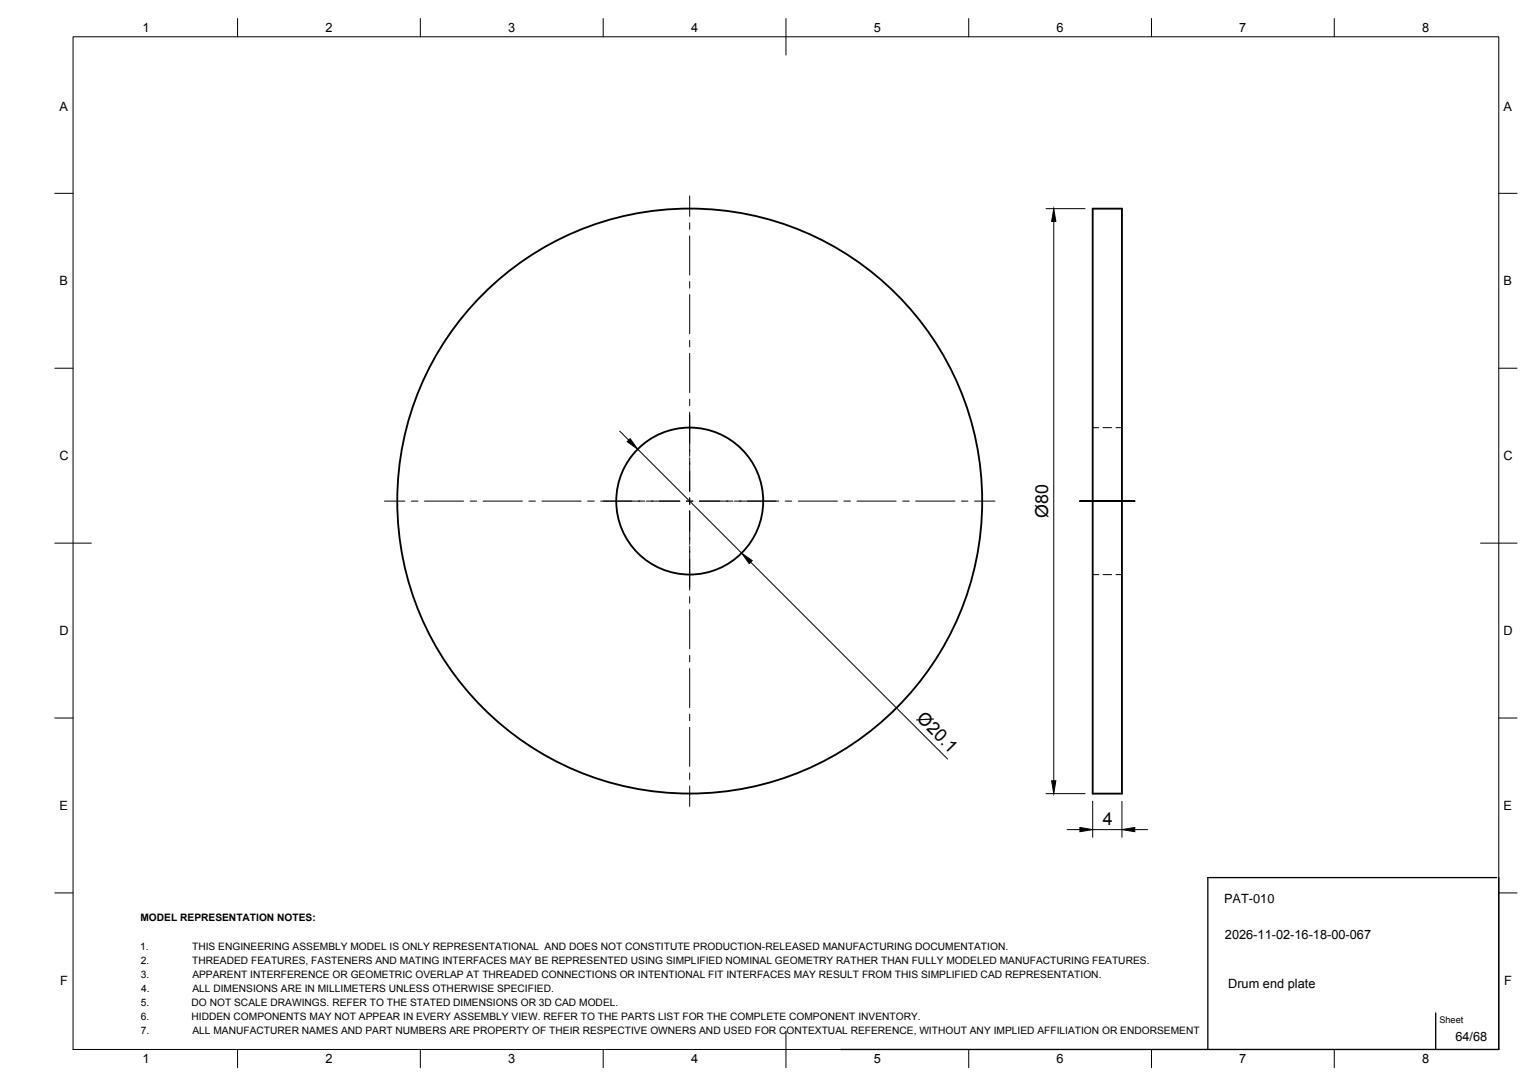
ISO-10303-21;
HEADER;
/* Generated by software containing ST-Developer
 * from STEP Tools, Inc. (www.steptools.com) 
 */

FILE_DESCRIPTION(
/* description */ ('Belt conveyor head drive unit'),
/* implementation_level */ '2;1');

FILE_NAME(
/* name */ 'Drum end plate.step',
/* time_stamp */ '2026-10-28T03:26:19-07:00',
/* author */ (''),
/* organization */ (''),
/* preprocessor_version */ 'ST-DEVELOPER v20.2',
/* originating_system */ 'Autodesk Translation Framework v15.17.0.0',
/* authorisation */ '');

FILE_SCHEMA (('AUTOMOTIVE_DESIGN { 1 0 10303 214 3 1 1 }'));
ENDSEC;

DATA;
#10=MECHANICAL_DESIGN_GEOMETRIC_PRESENTATION_REPRESENTATION('',(#925),#27069);
#771=SHAPE_REPRESENTATION_RELATIONSHIP('SRR','None',#27420,#840);
#840=ADVANCED_BREP_SHAPE_REPRESENTATION('',(#1006),#27062);
#925=STYLED_ITEM('',(#27790),#1006);
#1006=MANIFOLD_SOLID_BREP('Body1',#13794);
#1252=FACE_BOUND('',#3332,.T.);
#1253=FACE_BOUND('',#3334,.T.);
#1596=PLANE('',#15975);
#1597=PLANE('',#15976);
#2289=FACE_OUTER_BOUND('',#3329,.T.);
#2290=FACE_OUTER_BOUND('',#3330,.T.);
#2291=FACE_OUTER_BOUND('',#3331,.T.);
#2292=FACE_OUTER_BOUND('',#3333,.T.);
#3329=EDGE_LOOP('',(#11770,#11771,#11772,#11773));
#3330=EDGE_LOOP('',(#11774,#11775,#11776,#11777));
#3331=EDGE_LOOP('',(#11778));
#3332=EDGE_LOOP('',(#11779));
#3333=EDGE_LOOP('',(#11780));
#3334=EDGE_LOOP('',(#11781));
#4141=LINE('',#25622,#4933);
#4142=LINE('',#25628,#4934);
#4933=VECTOR('',#19895,1.005);
#4934=VECTOR('',#19902,4.);
#5751=CIRCLE('',#15970,1.005);
#5752=CIRCLE('',#15971,1.005);
#5753=CIRCLE('',#15973,4.);
#5754=CIRCLE('',#15974,4.);
#6915=VERTEX_POINT('',#25619);
#6916=VERTEX_POINT('',#25621);
#6917=VERTEX_POINT('',#25625);
#6918=VERTEX_POINT('',#25627);
#8577=EDGE_CURVE('',#6915,#6915,#5751,.T.);
#8578=EDGE_CURVE('',#6915,#6916,#4141,.T.);
#8579=EDGE_CURVE('',#6916,#6916,#5752,.T.);
#8580=EDGE_CURVE('',#6917,#6917,#5753,.T.);
#8581=EDGE_CURVE('',#6917,#6918,#4142,.T.);
#8582=EDGE_CURVE('',#6918,#6918,#5754,.T.);
#11770=ORIENTED_EDGE('',*,*,#8577,.F.);
#11771=ORIENTED_EDGE('',*,*,#8578,.T.);
#11772=ORIENTED_EDGE('',*,*,#8579,.T.);
#11773=ORIENTED_EDGE('',*,*,#8578,.F.);
#11774=ORIENTED_EDGE('',*,*,#8580,.F.);
#11775=ORIENTED_EDGE('',*,*,#8581,.T.);
#11776=ORIENTED_EDGE('',*,*,#8582,.T.);
#11777=ORIENTED_EDGE('',*,*,#8581,.F.);
#11778=ORIENTED_EDGE('',*,*,#8580,.T.);
#11779=ORIENTED_EDGE('',*,*,#8577,.T.);
#11780=ORIENTED_EDGE('',*,*,#8582,.F.);
#11781=ORIENTED_EDGE('',*,*,#8579,.F.);
#12811=CYLINDRICAL_SURFACE('',#15969,1.005);
#12812=CYLINDRICAL_SURFACE('',#15972,4.);
#13568=ADVANCED_FACE('',(#2289),#12811,.F.);
#13569=ADVANCED_FACE('',(#2290),#12812,.T.);
#13570=ADVANCED_FACE('',(#2291,#1252),#1596,.T.);
#13571=ADVANCED_FACE('',(#2292,#1253),#1597,.F.);
#13794=CLOSED_SHELL('',(#13568,#13569,#13570,#13571));
#15968=AXIS2_PLACEMENT_3D('',#25617,#19889,#19890);
#15969=AXIS2_PLACEMENT_3D('',#25618,#19891,#19892);
#15970=AXIS2_PLACEMENT_3D('',#25620,#19893,#19894);
#15971=AXIS2_PLACEMENT_3D('',#25623,#19896,#19897);
#15972=AXIS2_PLACEMENT_3D('',#25624,#19898,#19899);
#15973=AXIS2_PLACEMENT_3D('',#25626,#19900,#19901);
#15974=AXIS2_PLACEMENT_3D('',#25629,#19903,#19904);
#15975=AXIS2_PLACEMENT_3D('',#25630,#19905,#19906);
#15976=AXIS2_PLACEMENT_3D('',#25631,#19907,#19908);
#19889=DIRECTION('axis',(0.,0.,1.));
#19890=DIRECTION('refdir',(1.,0.,0.));
#19891=DIRECTION('center_axis',(0.,1.,0.));
#19892=DIRECTION('ref_axis',(1.,0.,0.));
#19893=DIRECTION('center_axis',(0.,-1.,0.));
#19894=DIRECTION('ref_axis',(1.,0.,0.));
#19895=DIRECTION('',(0.,-1.,0.));
#19896=DIRECTION('center_axis',(0.,-1.,0.));
#19897=DIRECTION('ref_axis',(1.,0.,0.));
#19898=DIRECTION('center_axis',(0.,1.,0.));
#19899=DIRECTION('ref_axis',(1.,0.,0.));
#19900=DIRECTION('center_axis',(0.,1.,0.));
#19901=DIRECTION('ref_axis',(1.,0.,0.));
#19902=DIRECTION('',(0.,-1.,0.));
#19903=DIRECTION('center_axis',(0.,1.,0.));
#19904=DIRECTION('ref_axis',(1.,0.,0.));
#19905=DIRECTION('center_axis',(0.,1.,0.));
#19906=DIRECTION('ref_axis',(1.,0.,0.));
#19907=DIRECTION('center_axis',(0.,1.,0.));
#19908=DIRECTION('ref_axis',(1.,0.,0.));
#25617=CARTESIAN_POINT('',(0.,0.,0.));
#25618=CARTESIAN_POINT('Origin',(6.97091003018116,6.6,7.));
#25619=CARTESIAN_POINT('',(5.96591003018116,7.,7.));
#25620=CARTESIAN_POINT('Origin',(6.97091003018116,7.,7.));
#25621=CARTESIAN_POINT('',(5.96591003018116,6.6,7.));
#25622=CARTESIAN_POINT('',(5.96591003018116,6.6,7.));
#25623=CARTESIAN_POINT('Origin',(6.97091003018116,6.6,7.));
#25624=CARTESIAN_POINT('Origin',(6.97091003018116,6.6,7.));
#25625=CARTESIAN_POINT('',(2.97091003018116,7.,7.));
#25626=CARTESIAN_POINT('Origin',(6.97091003018116,7.,7.));
#25627=CARTESIAN_POINT('',(2.97091003018116,6.6,7.));
#25628=CARTESIAN_POINT('',(2.97091003018116,6.6,7.));
#25629=CARTESIAN_POINT('Origin',(6.97091003018116,6.6,7.));
#25630=CARTESIAN_POINT('Origin',(6.97091003018116,7.,7.));
#25631=CARTESIAN_POINT('Origin',(6.97091003018116,6.6,7.));
#26985=UNCERTAINTY_MEASURE_WITH_UNIT(LENGTH_MEASURE(0.001),#27070,
'DISTANCE_ACCURACY_VALUE',
'Maximum model space distance between geometric entities at asserted c
onnectivities');
#26992=UNCERTAINTY_MEASURE_WITH_UNIT(LENGTH_MEASURE(0.001),#27070,
'DISTANCE_ACCURACY_VALUE',
'Maximum model space distance between geometric entities at asserted c
onnectivities');
#27062=(
GEOMETRIC_REPRESENTATION_CONTEXT(3)
GLOBAL_UNCERTAINTY_ASSIGNED_CONTEXT((#26985))
GLOBAL_UNIT_ASSIGNED_CONTEXT((#27070,#27072,#27073))
REPRESENTATION_CONTEXT('','3D')
);
#27069=(
GEOMETRIC_REPRESENTATION_CONTEXT(3)
GLOBAL_UNCERTAINTY_ASSIGNED_CONTEXT((#26992))
GLOBAL_UNIT_ASSIGNED_CONTEXT((#27070,#27072,#27073))
REPRESENTATION_CONTEXT('','3D')
);
#27070=(
LENGTH_UNIT()
NAMED_UNIT(*)
SI_UNIT(.CENTI.,.METRE.)
);
#27072=(
NAMED_UNIT(*)
PLANE_ANGLE_UNIT()
SI_UNIT($,.RADIAN.)
);
#27073=(
NAMED_UNIT(*)
SI_UNIT($,.STERADIAN.)
SOLID_ANGLE_UNIT()
);
#27143=SHAPE_DEFINITION_REPRESENTATION(#27231,#27420);
#27231=PRODUCT_DEFINITION_SHAPE('',$,#27497);
#27420=SHAPE_REPRESENTATION('',(#15968),#27062);
#27427=PRODUCT_DEFINITION_CONTEXT('part definition',#27657,'design');
#27497=PRODUCT_DEFINITION('Drum end plate','Drum end plate',#27573,#27427);
#27573=PRODUCT_DEFINITION_FORMATION('',$,#27728);
#27657=APPLICATION_CONTEXT(
'Core Data for Automotive Mechanical Design Process');
#27658=PRODUCT_CONTEXT('part definition',#27657,'mechanical');
#27728=PRODUCT('Drum end plate','Drum end plate','Drum end plate',(#27658));
#27784=COLOUR_RGB('Sky Blue',0.24,0.69,0.87);
#27785=FILL_AREA_STYLE_COLOUR('',#27784);
#27786=FILL_AREA_STYLE('',(#27785));
#27787=SURFACE_STYLE_FILL_AREA(#27786);
#27788=SURFACE_SIDE_STYLE('',(#27787));
#27789=SURFACE_STYLE_USAGE(.BOTH.,#27788);
#27790=PRESENTATION_STYLE_ASSIGNMENT((#27789));
ENDSEC;
END-ISO-10303-21;
